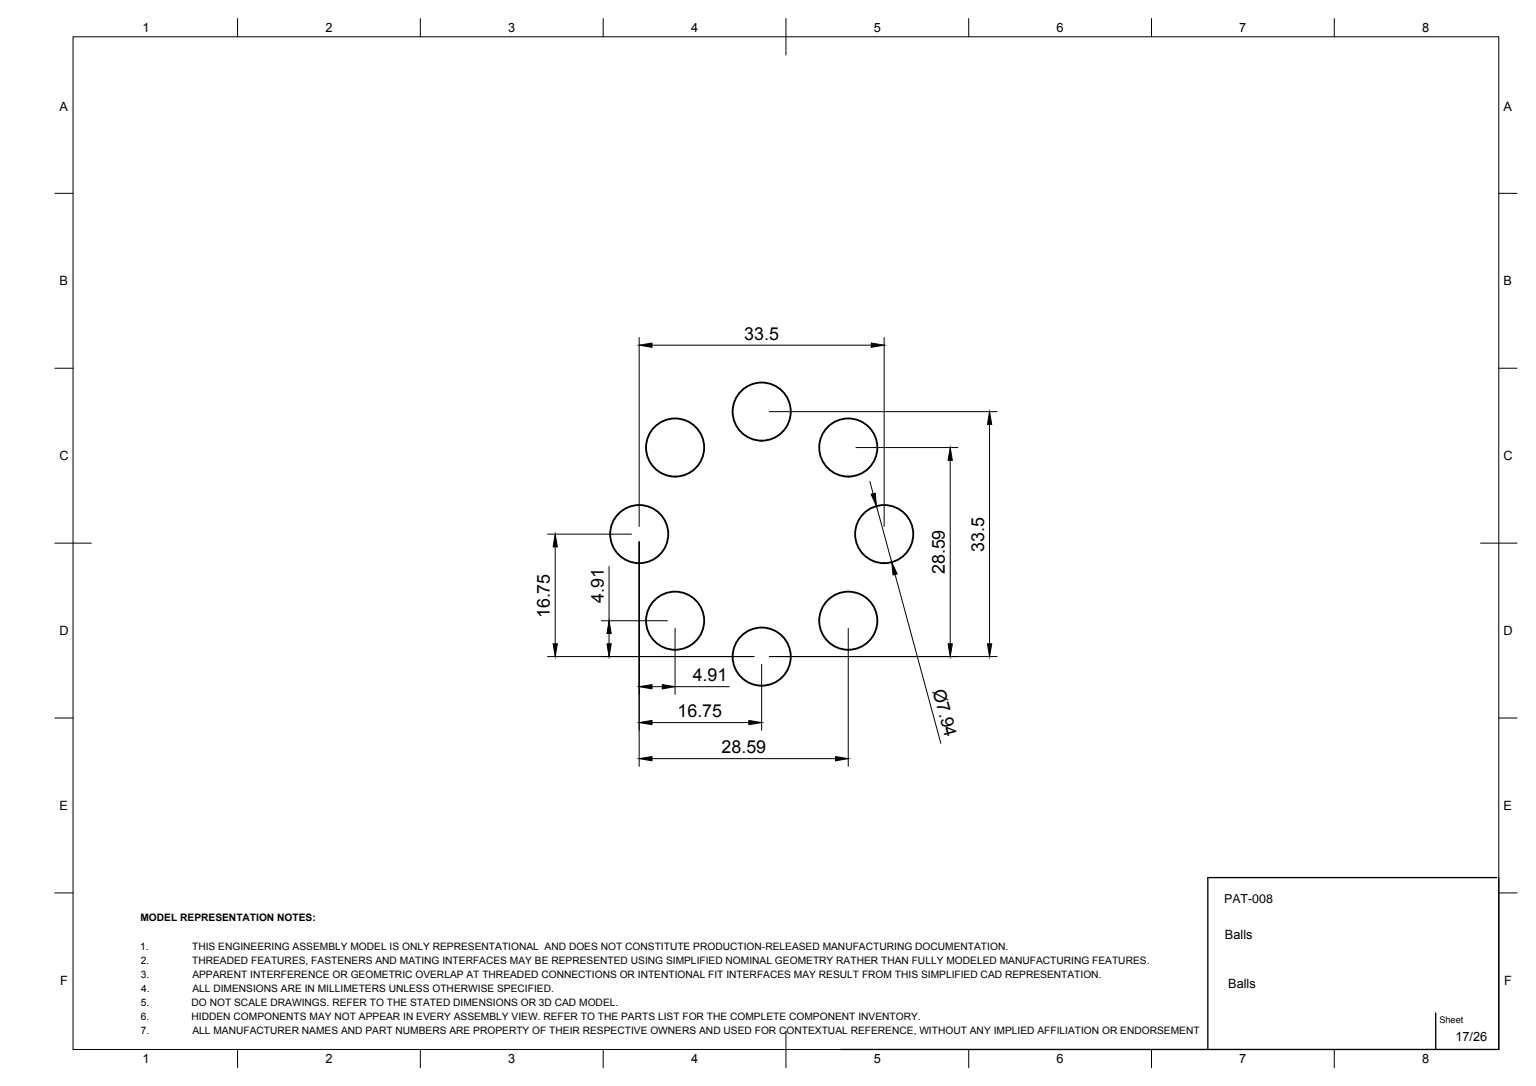
ISO-10303-21;
HEADER;
/* Generated by software containing ST-Developer
 * from STEP Tools, Inc. (www.steptools.com) 
 */

FILE_DESCRIPTION(
/* description */ ('Bearing housing with oil seal and end cap'),
/* implementation_level */ '2;1');

FILE_NAME(
/* name */ 'Balls.step',
/* time_stamp */ '2026-10-28T03:23:10-07:00',
/* author */ (''),
/* organization */ (''),
/* preprocessor_version */ 'ST-DEVELOPER v20.2',
/* originating_system */ 'Autodesk Translation Framework v15.17.0.0',
/* authorisation */ '');

FILE_SCHEMA (('AUTOMOTIVE_DESIGN { 1 0 10303 214 3 1 1 }'));
ENDSEC;

DATA;
#10=MECHANICAL_DESIGN_GEOMETRIC_PRESENTATION_REPRESENTATION('',(#269,#270,#271,#272,#273,#274,#275,#276),#7871);
#185=SPHERICAL_SURFACE('',#4597,0.3969);
#186=SPHERICAL_SURFACE('',#4599,0.3969);
#187=SPHERICAL_SURFACE('',#4601,0.3969);
#188=SPHERICAL_SURFACE('',#4603,0.3969);
#189=SPHERICAL_SURFACE('',#4605,0.3969);
#190=SPHERICAL_SURFACE('',#4607,0.3969);
#191=SPHERICAL_SURFACE('',#4609,0.3969);
#192=SPHERICAL_SURFACE('',#4611,0.3969);
#227=SHAPE_REPRESENTATION_RELATIONSHIP('SRR','None',#7975,#248);
#248=ADVANCED_BREP_SHAPE_REPRESENTATION('',(#298,#299,#300,#301,#302,#303,
#304,#305),#7859);
#269=STYLED_ITEM('',(#8153),#298);
#270=STYLED_ITEM('',(#8153),#299);
#271=STYLED_ITEM('',(#8153),#300);
#272=STYLED_ITEM('',(#8153),#301);
#273=STYLED_ITEM('',(#8153),#302);
#274=STYLED_ITEM('',(#8153),#303);
#275=STYLED_ITEM('',(#8153),#304);
#276=STYLED_ITEM('',(#8153),#305);
#298=MANIFOLD_SOLID_BREP('Body1',#4095);
#299=MANIFOLD_SOLID_BREP('Body2',#4096);
#300=MANIFOLD_SOLID_BREP('Body3',#4097);
#301=MANIFOLD_SOLID_BREP('Body4',#4098);
#302=MANIFOLD_SOLID_BREP('Body5',#4099);
#303=MANIFOLD_SOLID_BREP('Body6',#4100);
#304=MANIFOLD_SOLID_BREP('Body7',#4101);
#305=MANIFOLD_SOLID_BREP('Body8',#4102);
#673=FACE_OUTER_BOUND('',#987,.T.);
#674=FACE_OUTER_BOUND('',#988,.T.);
#675=FACE_OUTER_BOUND('',#989,.T.);
#676=FACE_OUTER_BOUND('',#990,.T.);
#677=FACE_OUTER_BOUND('',#991,.T.);
#678=FACE_OUTER_BOUND('',#992,.T.);
#679=FACE_OUTER_BOUND('',#993,.T.);
#680=FACE_OUTER_BOUND('',#994,.T.);
#987=EDGE_LOOP('',(#3219,#3220));
#988=EDGE_LOOP('',(#3221,#3222));
#989=EDGE_LOOP('',(#3223,#3224));
#990=EDGE_LOOP('',(#3225,#3226));
#991=EDGE_LOOP('',(#3227,#3228));
#992=EDGE_LOOP('',(#3229,#3230));
#993=EDGE_LOOP('',(#3231,#3232));
#994=EDGE_LOOP('',(#3233,#3234));
#1785=CIRCLE('',#4598,0.3969);
#1786=CIRCLE('',#4600,0.3969);
#1787=CIRCLE('',#4602,0.3969);
#1788=CIRCLE('',#4604,0.3969);
#1789=CIRCLE('',#4606,0.3969);
#1790=CIRCLE('',#4608,0.3969);
#1791=CIRCLE('',#4610,0.3969);
#1792=CIRCLE('',#4612,0.3969);
#2047=VERTEX_POINT('',#6736);
#2048=VERTEX_POINT('',#6737);
#2049=VERTEX_POINT('',#6740);
#2050=VERTEX_POINT('',#6741);
#2051=VERTEX_POINT('',#6744);
#2052=VERTEX_POINT('',#6745);
#2053=VERTEX_POINT('',#6748);
#2054=VERTEX_POINT('',#6749);
#2055=VERTEX_POINT('',#6752);
#2056=VERTEX_POINT('',#6753);
#2057=VERTEX_POINT('',#6756);
#2058=VERTEX_POINT('',#6757);
#2059=VERTEX_POINT('',#6760);
#2060=VERTEX_POINT('',#6761);
#2061=VERTEX_POINT('',#6764);
#2062=VERTEX_POINT('',#6765);
#2473=EDGE_CURVE('',#2047,#2048,#1785,.T.);
#2474=EDGE_CURVE('',#2049,#2050,#1786,.T.);
#2475=EDGE_CURVE('',#2051,#2052,#1787,.T.);
#2476=EDGE_CURVE('',#2053,#2054,#1788,.T.);
#2477=EDGE_CURVE('',#2055,#2056,#1789,.T.);
#2478=EDGE_CURVE('',#2057,#2058,#1790,.T.);
#2479=EDGE_CURVE('',#2059,#2060,#1791,.T.);
#2480=EDGE_CURVE('',#2061,#2062,#1792,.T.);
#3219=ORIENTED_EDGE('',*,*,#2473,.T.);
#3220=ORIENTED_EDGE('',*,*,#2473,.F.);
#3221=ORIENTED_EDGE('',*,*,#2474,.T.);
#3222=ORIENTED_EDGE('',*,*,#2474,.F.);
#3223=ORIENTED_EDGE('',*,*,#2475,.T.);
#3224=ORIENTED_EDGE('',*,*,#2475,.F.);
#3225=ORIENTED_EDGE('',*,*,#2476,.T.);
#3226=ORIENTED_EDGE('',*,*,#2476,.F.);
#3227=ORIENTED_EDGE('',*,*,#2477,.T.);
#3228=ORIENTED_EDGE('',*,*,#2477,.F.);
#3229=ORIENTED_EDGE('',*,*,#2478,.T.);
#3230=ORIENTED_EDGE('',*,*,#2478,.F.);
#3231=ORIENTED_EDGE('',*,*,#2479,.T.);
#3232=ORIENTED_EDGE('',*,*,#2479,.F.);
#3233=ORIENTED_EDGE('',*,*,#2480,.T.);
#3234=ORIENTED_EDGE('',*,*,#2480,.F.);
#3955=ADVANCED_FACE('',(#673),#185,.T.);
#3956=ADVANCED_FACE('',(#674),#186,.T.);
#3957=ADVANCED_FACE('',(#675),#187,.T.);
#3958=ADVANCED_FACE('',(#676),#188,.T.);
#3959=ADVANCED_FACE('',(#677),#189,.T.);
#3960=ADVANCED_FACE('',(#678),#190,.T.);
#3961=ADVANCED_FACE('',(#679),#191,.T.);
#3962=ADVANCED_FACE('',(#680),#192,.T.);
#4095=CLOSED_SHELL('',(#3955));
#4096=CLOSED_SHELL('',(#3956));
#4097=CLOSED_SHELL('',(#3957));
#4098=CLOSED_SHELL('',(#3958));
#4099=CLOSED_SHELL('',(#3959));
#4100=CLOSED_SHELL('',(#3960));
#4101=CLOSED_SHELL('',(#3961));
#4102=CLOSED_SHELL('',(#3962));
#4596=AXIS2_PLACEMENT_3D('',#6734,#5500,#5501);
#4597=AXIS2_PLACEMENT_3D('',#6735,#5502,#5503);
#4598=AXIS2_PLACEMENT_3D('',#6738,#5504,#5505);
#4599=AXIS2_PLACEMENT_3D('',#6739,#5506,#5507);
#4600=AXIS2_PLACEMENT_3D('',#6742,#5508,#5509);
#4601=AXIS2_PLACEMENT_3D('',#6743,#5510,#5511);
#4602=AXIS2_PLACEMENT_3D('',#6746,#5512,#5513);
#4603=AXIS2_PLACEMENT_3D('',#6747,#5514,#5515);
#4604=AXIS2_PLACEMENT_3D('',#6750,#5516,#5517);
#4605=AXIS2_PLACEMENT_3D('',#6751,#5518,#5519);
#4606=AXIS2_PLACEMENT_3D('',#6754,#5520,#5521);
#4607=AXIS2_PLACEMENT_3D('',#6755,#5522,#5523);
#4608=AXIS2_PLACEMENT_3D('',#6758,#5524,#5525);
#4609=AXIS2_PLACEMENT_3D('',#6759,#5526,#5527);
#4610=AXIS2_PLACEMENT_3D('',#6762,#5528,#5529);
#4611=AXIS2_PLACEMENT_3D('',#6763,#5530,#5531);
#4612=AXIS2_PLACEMENT_3D('',#6766,#5532,#5533);
#5500=DIRECTION('axis',(0.,0.,1.));
#5501=DIRECTION('refdir',(1.,0.,0.));
#5502=DIRECTION('center_axis',(0.,0.,1.));
#5503=DIRECTION('ref_axis',(1.,0.,0.));
#5504=DIRECTION('center_axis',(1.22464679914735E-16,-1.,0.));
#5505=DIRECTION('ref_axis',(-1.,-1.22464679914735E-16,0.));
#5506=DIRECTION('center_axis',(0.707106781186548,0.,0.707106781186548));
#5507=DIRECTION('ref_axis',(0.707106781186548,0.,-0.707106781186548));
#5508=DIRECTION('center_axis',(8.65956056235493E-17,-1.,-8.65956056235493E-17));
#5509=DIRECTION('ref_axis',(-0.707106781186548,-1.22464679914735E-16,0.707106781186548));
#5510=DIRECTION('center_axis',(1.,0.,0.));
#5511=DIRECTION('ref_axis',(6.12323399573677E-17,0.,-1.));
#5512=DIRECTION('center_axis',(7.49879891330929E-33,-1.,-1.22464679914735E-16));
#5513=DIRECTION('ref_axis',(-6.12323399573677E-17,-1.22464679914735E-16,
1.));
#5514=DIRECTION('center_axis',(0.707106781186548,0.,-0.707106781186548));
#5515=DIRECTION('ref_axis',(-0.707106781186548,0.,-0.707106781186548));
#5516=DIRECTION('center_axis',(-8.65956056235493E-17,-1.,-8.65956056235493E-17));
#5517=DIRECTION('ref_axis',(0.707106781186548,-1.22464679914735E-16,0.707106781186548));
#5518=DIRECTION('center_axis',(0.,0.,-1.));
#5519=DIRECTION('ref_axis',(-1.,0.,-1.22464679914735E-16));
#5520=DIRECTION('center_axis',(-1.22464679914735E-16,-1.,-1.49975978266186E-32));
#5521=DIRECTION('ref_axis',(1.,-1.22464679914735E-16,1.22464679914735E-16));
#5522=DIRECTION('center_axis',(-0.707106781186548,0.,-0.707106781186548));
#5523=DIRECTION('ref_axis',(-0.707106781186548,0.,0.707106781186548));
#5524=DIRECTION('center_axis',(-8.65956056235493E-17,-1.,8.65956056235493E-17));
#5525=DIRECTION('ref_axis',(0.707106781186548,-1.22464679914735E-16,-0.707106781186548));
#5526=DIRECTION('center_axis',(-1.,0.,0.));
#5527=DIRECTION('ref_axis',(-1.83697019872103E-16,0.,1.));
#5528=DIRECTION('center_axis',(-2.24963967399279E-32,-1.,1.22464679914735E-16));
#5529=DIRECTION('ref_axis',(1.83697019872103E-16,-1.22464679914735E-16,
-1.));
#5530=DIRECTION('center_axis',(-0.707106781186548,0.,0.707106781186548));
#5531=DIRECTION('ref_axis',(0.707106781186548,0.,0.707106781186548));
#5532=DIRECTION('center_axis',(8.65956056235493E-17,-1.,8.65956056235494E-17));
#5533=DIRECTION('ref_axis',(-0.707106781186548,-1.22464679914735E-16,-0.707106781186548));
#6734=CARTESIAN_POINT('',(0.,0.,0.));
#6735=CARTESIAN_POINT('Origin',(1.675,0.,0.));
#6736=CARTESIAN_POINT('',(1.675,-2.97627328869245E-33,0.3969));
#6737=CARTESIAN_POINT('',(1.675,-2.97627328869245E-33,-0.3969));
#6738=CARTESIAN_POINT('Origin',(1.675,0.,0.));
#6739=CARTESIAN_POINT('Origin',(1.18440385848747,0.,-1.18440385848747));
#6740=CARTESIAN_POINT('',(1.46505453994041,3.1867025333467E-33,-0.903753177034526));
#6741=CARTESIAN_POINT('',(0.903753177034527,-9.13924911073161E-33,-1.46505453994041));
#6742=CARTESIAN_POINT('Origin',(1.18440385848747,0.,-1.18440385848747));
#6743=CARTESIAN_POINT('Origin',(1.02564169428591E-16,0.,-1.675));
#6744=CARTESIAN_POINT('',(0.3969,-2.97627328869246E-33,-1.675));
#6745=CARTESIAN_POINT('',(-0.3969,-2.97627328869245E-33,-1.675));
#6746=CARTESIAN_POINT('Origin',(1.02564169428591E-16,0.,-1.675));
#6747=CARTESIAN_POINT('Origin',(-1.18440385848747,0.,-1.18440385848747));
#6748=CARTESIAN_POINT('',(-0.903753177034526,3.1867025333467E-33,-1.46505453994041));
#6749=CARTESIAN_POINT('',(-1.46505453994041,-9.13924911073161E-33,-0.903753177034527));
#6750=CARTESIAN_POINT('Origin',(-1.18440385848747,0.,-1.18440385848747));
#6751=CARTESIAN_POINT('Origin',(-1.675,0.,-2.05128338857182E-16));
#6752=CARTESIAN_POINT('',(-1.675,-2.97627328869246E-33,-0.3969));
#6753=CARTESIAN_POINT('',(-1.675,-2.97627328869245E-33,0.3969));
#6754=CARTESIAN_POINT('Origin',(-1.675,0.,-2.05128338857182E-16));
#6755=CARTESIAN_POINT('Origin',(-1.18440385848747,0.,1.18440385848747));
#6756=CARTESIAN_POINT('',(-1.46505453994041,6.26819044436628E-33,0.903753177034526));
#6757=CARTESIAN_POINT('',(-0.903753177034527,-1.22207370217512E-32,1.46505453994041));
#6758=CARTESIAN_POINT('Origin',(-1.18440385848747,0.,1.18440385848747));
#6759=CARTESIAN_POINT('Origin',(-3.07692508285772E-16,0.,1.675));
#6760=CARTESIAN_POINT('',(-0.3969,-2.97627328869246E-33,1.675));
#6761=CARTESIAN_POINT('',(0.396899999999999,-2.97627328869245E-33,1.675));
#6762=CARTESIAN_POINT('Origin',(-3.07692508285772E-16,0.,1.675));
#6763=CARTESIAN_POINT('Origin',(1.18440385848747,0.,1.18440385848747));
#6764=CARTESIAN_POINT('',(0.903753177034526,9.34967835538585E-33,1.46505453994041));
#6765=CARTESIAN_POINT('',(1.46505453994041,-1.53022249327708E-32,0.903753177034527));
#6766=CARTESIAN_POINT('Origin',(1.18440385848747,0.,1.18440385848747));
#7833=UNCERTAINTY_MEASURE_WITH_UNIT(LENGTH_MEASURE(0.001),#7872,
'DISTANCE_ACCURACY_VALUE',
'Maximum model space distance between geometric entities at asserted c
onnectivities');
#7845=UNCERTAINTY_MEASURE_WITH_UNIT(LENGTH_MEASURE(0.001),#7872,
'DISTANCE_ACCURACY_VALUE',
'Maximum model space distance between geometric entities at asserted c
onnectivities');
#7859=(
GEOMETRIC_REPRESENTATION_CONTEXT(3)
GLOBAL_UNCERTAINTY_ASSIGNED_CONTEXT((#7833))
GLOBAL_UNIT_ASSIGNED_CONTEXT((#7872,#7874,#7875))
REPRESENTATION_CONTEXT('','3D')
);
#7871=(
GEOMETRIC_REPRESENTATION_CONTEXT(3)
GLOBAL_UNCERTAINTY_ASSIGNED_CONTEXT((#7845))
GLOBAL_UNIT_ASSIGNED_CONTEXT((#7872,#7874,#7875))
REPRESENTATION_CONTEXT('','3D')
);
#7872=(
LENGTH_UNIT()
NAMED_UNIT(*)
SI_UNIT(.CENTI.,.METRE.)
);
#7874=(
NAMED_UNIT(*)
PLANE_ANGLE_UNIT()
SI_UNIT($,.RADIAN.)
);
#7875=(
NAMED_UNIT(*)
SI_UNIT($,.STERADIAN.)
SOLID_ANGLE_UNIT()
);
#7889=SHAPE_DEFINITION_REPRESENTATION(#7914,#7975);
#7914=PRODUCT_DEFINITION_SHAPE('',$,#8001);
#7975=SHAPE_REPRESENTATION('',(#4596),#7859);
#7987=PRODUCT_DEFINITION_CONTEXT('part definition',#8064,'design');
#8001=PRODUCT_DEFINITION('Balls','Balls',#8026,#7987);
#8026=PRODUCT_DEFINITION_FORMATION('',$,#8079);
#8064=APPLICATION_CONTEXT(
'Core Data for Automotive Mechanical Design Process');
#8065=PRODUCT_CONTEXT('part definition',#8064,'mechanical');
#8079=PRODUCT('Balls','Balls','Balls',(#8065));
#8147=COLOUR_RGB('Grey',0.48,0.52,0.57);
#8148=FILL_AREA_STYLE_COLOUR('',#8147);
#8149=FILL_AREA_STYLE('',(#8148));
#8150=SURFACE_STYLE_FILL_AREA(#8149);
#8151=SURFACE_SIDE_STYLE('',(#8150));
#8152=SURFACE_STYLE_USAGE(.BOTH.,#8151);
#8153=PRESENTATION_STYLE_ASSIGNMENT((#8152));
ENDSEC;
END-ISO-10303-21;
